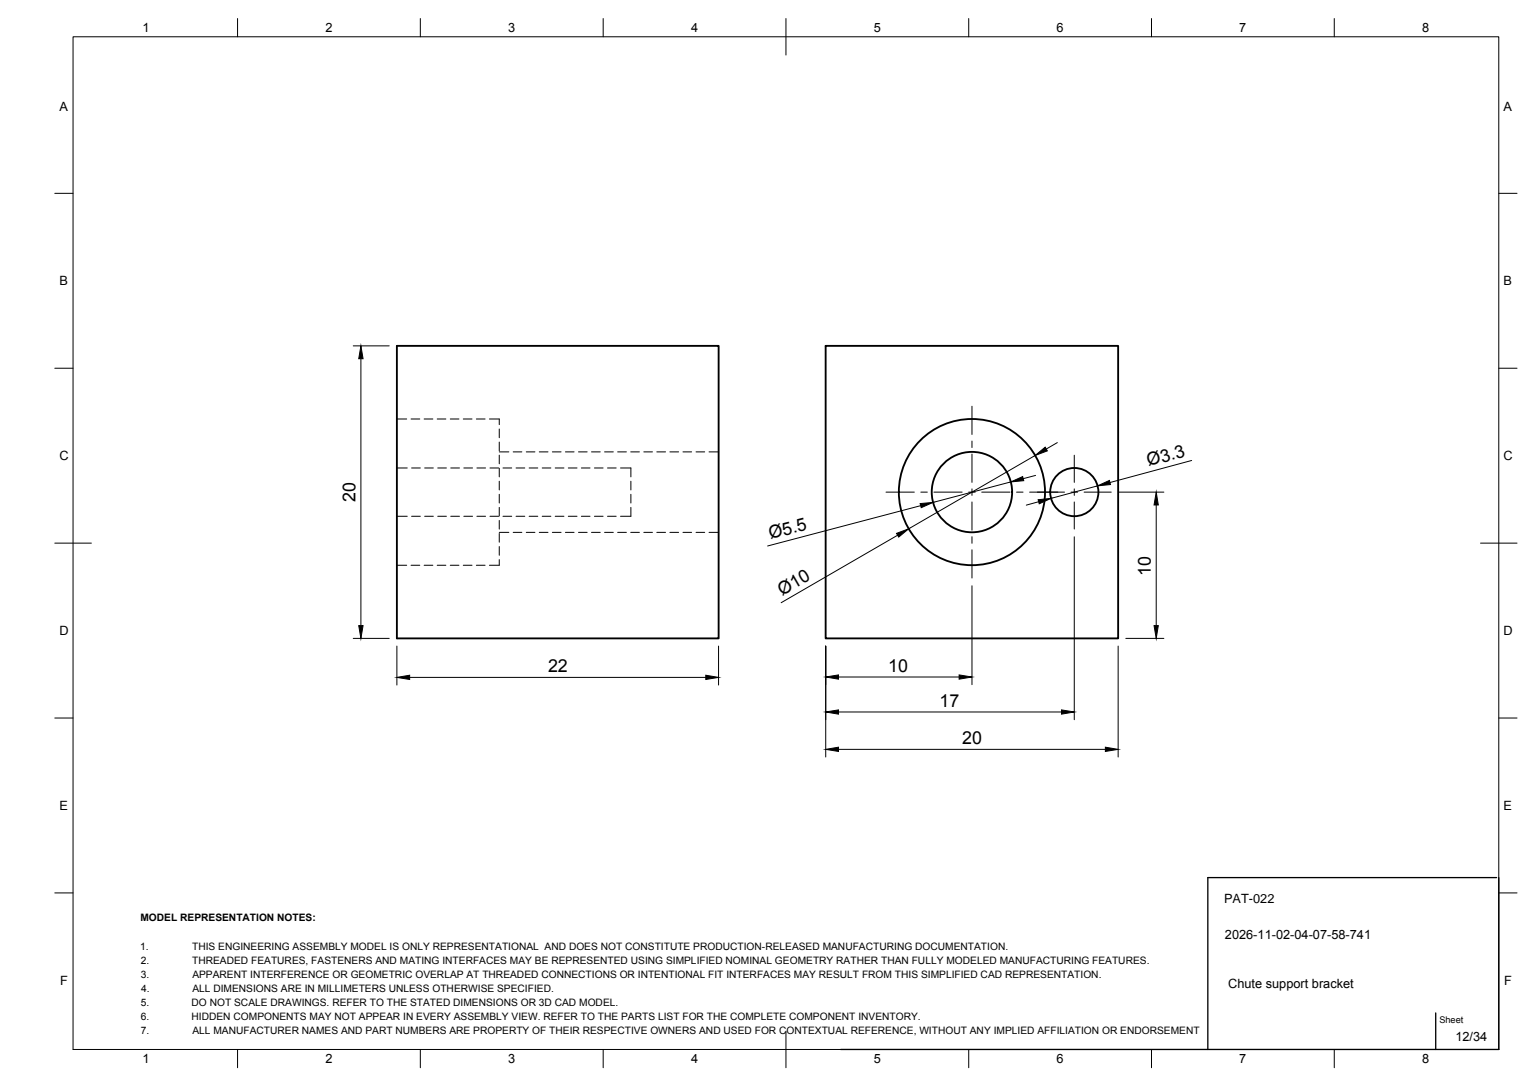
ISO-10303-21;
HEADER;
/* Generated by software containing ST-Developer
 * from STEP Tools, Inc. (www.steptools.com) 
 */

FILE_DESCRIPTION(
/* description */ ('Chute with adjustable gate'),
/* implementation_level */ '2;1');

FILE_NAME(
/* name */ 'Chute support bracket.step',
/* time_stamp */ '2026-10-27T10:52:28-07:00',
/* author */ (''),
/* organization */ (''),
/* preprocessor_version */ 'ST-DEVELOPER v20.2',
/* originating_system */ 'Autodesk Translation Framework v15.17.0.0',
/* authorisation */ '');

FILE_SCHEMA (('AUTOMOTIVE_DESIGN { 1 0 10303 214 3 1 1 }'));
ENDSEC;

DATA;
#10=MECHANICAL_DESIGN_GEOMETRIC_PRESENTATION_REPRESENTATION('',(#421),#13094);
#357=SHAPE_REPRESENTATION_RELATIONSHIP('SRR','None',#13258,#389);
#389=ADVANCED_BREP_SHAPE_REPRESENTATION('',(#453),#13067);
#421=STYLED_ITEM('',(#13474),#453);
#453=MANIFOLD_SOLID_BREP('Body1',#7604);
#500=FACE_BOUND('',#1417,.T.);
#501=FACE_BOUND('',#1420,.T.);
#502=FACE_BOUND('',#1421,.T.);
#503=FACE_BOUND('',#1424,.T.);
#636=PLANE('',#8081);
#637=PLANE('',#8085);
#638=PLANE('',#8089);
#639=PLANE('',#8090);
#640=PLANE('',#8091);
#641=PLANE('',#8092);
#642=PLANE('',#8093);
#643=PLANE('',#8094);
#972=FACE_OUTER_BOUND('',#1413,.T.);
#973=FACE_OUTER_BOUND('',#1414,.T.);
#974=FACE_OUTER_BOUND('',#1415,.T.);
#975=FACE_OUTER_BOUND('',#1416,.T.);
#976=FACE_OUTER_BOUND('',#1418,.T.);
#977=FACE_OUTER_BOUND('',#1419,.T.);
#978=FACE_OUTER_BOUND('',#1422,.T.);
#979=FACE_OUTER_BOUND('',#1423,.T.);
#980=FACE_OUTER_BOUND('',#1425,.T.);
#981=FACE_OUTER_BOUND('',#1426,.T.);
#982=FACE_OUTER_BOUND('',#1427,.T.);
#1413=EDGE_LOOP('',(#5450,#5451,#5452,#5453));
#1414=EDGE_LOOP('',(#5454));
#1415=EDGE_LOOP('',(#5455,#5456,#5457,#5458));
#1416=EDGE_LOOP('',(#5459));
#1417=EDGE_LOOP('',(#5460));
#1418=EDGE_LOOP('',(#5461,#5462,#5463,#5464));
#1419=EDGE_LOOP('',(#5465,#5466,#5467,#5468));
#1420=EDGE_LOOP('',(#5469));
#1421=EDGE_LOOP('',(#5470));
#1422=EDGE_LOOP('',(#5471,#5472,#5473,#5474));
#1423=EDGE_LOOP('',(#5475,#5476,#5477,#5478));
#1424=EDGE_LOOP('',(#5479));
#1425=EDGE_LOOP('',(#5480,#5481,#5482,#5483));
#1426=EDGE_LOOP('',(#5484,#5485,#5486,#5487));
#1427=EDGE_LOOP('',(#5488,#5489,#5490,#5491));
#1968=LINE('',#11191,#2745);
#1969=LINE('',#11198,#2746);
#1970=LINE('',#11206,#2747);
#1971=LINE('',#11210,#2748);
#1972=LINE('',#11212,#2749);
#1973=LINE('',#11214,#2750);
#1974=LINE('',#11215,#2751);
#1975=LINE('',#11218,#2752);
#1976=LINE('',#11220,#2753);
#1977=LINE('',#11221,#2754);
#1978=LINE('',#11224,#2755);
#1979=LINE('',#11226,#2756);
#1980=LINE('',#11227,#2757);
#1981=LINE('',#11229,#2758);
#1982=LINE('',#11230,#2759);
#2745=VECTOR('',#8994,0.165);
#2746=VECTOR('',#9003,0.5);
#2747=VECTOR('',#9014,0.275);
#2748=VECTOR('',#9017,1.);
#2749=VECTOR('',#9018,1.);
#2750=VECTOR('',#9019,1.);
#2751=VECTOR('',#9020,1.);
#2752=VECTOR('',#9023,1.);
#2753=VECTOR('',#9024,1.);
#2754=VECTOR('',#9025,1.);
#2755=VECTOR('',#9028,1.);
#2756=VECTOR('',#9029,1.);
#2757=VECTOR('',#9030,1.);
#2758=VECTOR('',#9033,1.);
#2759=VECTOR('',#9034,1.);
#3438=CIRCLE('',#8079,0.165);
#3439=CIRCLE('',#8080,0.165);
#3440=CIRCLE('',#8083,0.5);
#3441=CIRCLE('',#8084,0.5);
#3442=CIRCLE('',#8086,0.275);
#3443=CIRCLE('',#8088,0.275);
#3681=VERTEX_POINT('',#11188);
#3682=VERTEX_POINT('',#11190);
#3683=VERTEX_POINT('',#11195);
#3684=VERTEX_POINT('',#11197);
#3685=VERTEX_POINT('',#11201);
#3686=VERTEX_POINT('',#11204);
#3687=VERTEX_POINT('',#11208);
#3688=VERTEX_POINT('',#11209);
#3689=VERTEX_POINT('',#11211);
#3690=VERTEX_POINT('',#11213);
#3691=VERTEX_POINT('',#11217);
#3692=VERTEX_POINT('',#11219);
#3693=VERTEX_POINT('',#11223);
#3694=VERTEX_POINT('',#11225);
#4358=EDGE_CURVE('',#3681,#3681,#3438,.T.);
#4359=EDGE_CURVE('',#3681,#3682,#1968,.T.);
#4360=EDGE_CURVE('',#3682,#3682,#3439,.T.);
#4361=EDGE_CURVE('',#3683,#3683,#3440,.T.);
#4362=EDGE_CURVE('',#3683,#3684,#1969,.T.);
#4363=EDGE_CURVE('',#3684,#3684,#3441,.T.);
#4364=EDGE_CURVE('',#3685,#3685,#3442,.T.);
#4365=EDGE_CURVE('',#3686,#3686,#3443,.T.);
#4366=EDGE_CURVE('',#3686,#3685,#1970,.T.);
#4367=EDGE_CURVE('',#3687,#3688,#1971,.T.);
#4368=EDGE_CURVE('',#3688,#3689,#1972,.T.);
#4369=EDGE_CURVE('',#3690,#3689,#1973,.T.);
#4370=EDGE_CURVE('',#3687,#3690,#1974,.T.);
#4371=EDGE_CURVE('',#3691,#3687,#1975,.T.);
#4372=EDGE_CURVE('',#3692,#3690,#1976,.T.);
#4373=EDGE_CURVE('',#3691,#3692,#1977,.T.);
#4374=EDGE_CURVE('',#3693,#3691,#1978,.T.);
#4375=EDGE_CURVE('',#3694,#3692,#1979,.T.);
#4376=EDGE_CURVE('',#3693,#3694,#1980,.T.);
#4377=EDGE_CURVE('',#3688,#3693,#1981,.T.);
#4378=EDGE_CURVE('',#3689,#3694,#1982,.T.);
#5450=ORIENTED_EDGE('',*,*,#4358,.F.);
#5451=ORIENTED_EDGE('',*,*,#4359,.T.);
#5452=ORIENTED_EDGE('',*,*,#4360,.F.);
#5453=ORIENTED_EDGE('',*,*,#4359,.F.);
#5454=ORIENTED_EDGE('',*,*,#4358,.T.);
#5455=ORIENTED_EDGE('',*,*,#4361,.F.);
#5456=ORIENTED_EDGE('',*,*,#4362,.T.);
#5457=ORIENTED_EDGE('',*,*,#4363,.F.);
#5458=ORIENTED_EDGE('',*,*,#4362,.F.);
#5459=ORIENTED_EDGE('',*,*,#4361,.T.);
#5460=ORIENTED_EDGE('',*,*,#4364,.F.);
#5461=ORIENTED_EDGE('',*,*,#4365,.F.);
#5462=ORIENTED_EDGE('',*,*,#4366,.T.);
#5463=ORIENTED_EDGE('',*,*,#4364,.T.);
#5464=ORIENTED_EDGE('',*,*,#4366,.F.);
#5465=ORIENTED_EDGE('',*,*,#4367,.T.);
#5466=ORIENTED_EDGE('',*,*,#4368,.T.);
#5467=ORIENTED_EDGE('',*,*,#4369,.F.);
#5468=ORIENTED_EDGE('',*,*,#4370,.F.);
#5469=ORIENTED_EDGE('',*,*,#4360,.T.);
#5470=ORIENTED_EDGE('',*,*,#4363,.T.);
#5471=ORIENTED_EDGE('',*,*,#4371,.T.);
#5472=ORIENTED_EDGE('',*,*,#4370,.T.);
#5473=ORIENTED_EDGE('',*,*,#4372,.F.);
#5474=ORIENTED_EDGE('',*,*,#4373,.F.);
#5475=ORIENTED_EDGE('',*,*,#4374,.T.);
#5476=ORIENTED_EDGE('',*,*,#4373,.T.);
#5477=ORIENTED_EDGE('',*,*,#4375,.F.);
#5478=ORIENTED_EDGE('',*,*,#4376,.F.);
#5479=ORIENTED_EDGE('',*,*,#4365,.T.);
#5480=ORIENTED_EDGE('',*,*,#4377,.T.);
#5481=ORIENTED_EDGE('',*,*,#4376,.T.);
#5482=ORIENTED_EDGE('',*,*,#4378,.F.);
#5483=ORIENTED_EDGE('',*,*,#4368,.F.);
#5484=ORIENTED_EDGE('',*,*,#4378,.T.);
#5485=ORIENTED_EDGE('',*,*,#4375,.T.);
#5486=ORIENTED_EDGE('',*,*,#4372,.T.);
#5487=ORIENTED_EDGE('',*,*,#4369,.T.);
#5488=ORIENTED_EDGE('',*,*,#4377,.F.);
#5489=ORIENTED_EDGE('',*,*,#4367,.F.);
#5490=ORIENTED_EDGE('',*,*,#4371,.F.);
#5491=ORIENTED_EDGE('',*,*,#4374,.F.);
#7118=CYLINDRICAL_SURFACE('',#8078,0.165);
#7119=CYLINDRICAL_SURFACE('',#8082,0.5);
#7120=CYLINDRICAL_SURFACE('',#8087,0.275);
#7240=ADVANCED_FACE('',(#972),#7118,.F.);
#7241=ADVANCED_FACE('',(#973),#636,.T.);
#7242=ADVANCED_FACE('',(#974),#7119,.F.);
#7243=ADVANCED_FACE('',(#975,#500),#637,.T.);
#7244=ADVANCED_FACE('',(#976),#7120,.F.);
#7245=ADVANCED_FACE('',(#977,#501,#502),#638,.T.);
#7246=ADVANCED_FACE('',(#978),#639,.T.);
#7247=ADVANCED_FACE('',(#979,#503),#640,.T.);
#7248=ADVANCED_FACE('',(#980),#641,.T.);
#7249=ADVANCED_FACE('',(#981),#642,.T.);
#7250=ADVANCED_FACE('',(#982),#643,.F.);
#7604=CLOSED_SHELL('',(#7240,#7241,#7242,#7243,#7244,#7245,#7246,#7247,
#7248,#7249,#7250));
#8077=AXIS2_PLACEMENT_3D('',#11186,#8988,#8989);
#8078=AXIS2_PLACEMENT_3D('',#11187,#8990,#8991);
#8079=AXIS2_PLACEMENT_3D('',#11189,#8992,#8993);
#8080=AXIS2_PLACEMENT_3D('',#11192,#8995,#8996);
#8081=AXIS2_PLACEMENT_3D('',#11193,#8997,#8998);
#8082=AXIS2_PLACEMENT_3D('',#11194,#8999,#9000);
#8083=AXIS2_PLACEMENT_3D('',#11196,#9001,#9002);
#8084=AXIS2_PLACEMENT_3D('',#11199,#9004,#9005);
#8085=AXIS2_PLACEMENT_3D('',#11200,#9006,#9007);
#8086=AXIS2_PLACEMENT_3D('',#11202,#9008,#9009);
#8087=AXIS2_PLACEMENT_3D('',#11203,#9010,#9011);
#8088=AXIS2_PLACEMENT_3D('',#11205,#9012,#9013);
#8089=AXIS2_PLACEMENT_3D('',#11207,#9015,#9016);
#8090=AXIS2_PLACEMENT_3D('',#11216,#9021,#9022);
#8091=AXIS2_PLACEMENT_3D('',#11222,#9026,#9027);
#8092=AXIS2_PLACEMENT_3D('',#11228,#9031,#9032);
#8093=AXIS2_PLACEMENT_3D('',#11231,#9035,#9036);
#8094=AXIS2_PLACEMENT_3D('',#11232,#9037,#9038);
#8988=DIRECTION('axis',(0.,0.,1.));
#8989=DIRECTION('refdir',(1.,0.,0.));
#8990=DIRECTION('center_axis',(0.,1.,0.));
#8991=DIRECTION('ref_axis',(1.,0.,0.));
#8992=DIRECTION('center_axis',(0.,1.,0.));
#8993=DIRECTION('ref_axis',(1.,0.,0.));
#8994=DIRECTION('',(0.,1.,0.));
#8995=DIRECTION('center_axis',(0.,-1.,0.));
#8996=DIRECTION('ref_axis',(1.,0.,0.));
#8997=DIRECTION('center_axis',(0.,1.,0.));
#8998=DIRECTION('ref_axis',(1.,0.,0.));
#8999=DIRECTION('center_axis',(0.,1.,0.));
#9000=DIRECTION('ref_axis',(1.,0.,0.));
#9001=DIRECTION('center_axis',(0.,1.,0.));
#9002=DIRECTION('ref_axis',(1.,0.,0.));
#9003=DIRECTION('',(0.,1.,0.));
#9004=DIRECTION('center_axis',(0.,-1.,0.));
#9005=DIRECTION('ref_axis',(1.,0.,0.));
#9006=DIRECTION('center_axis',(0.,1.,0.));
#9007=DIRECTION('ref_axis',(1.,0.,0.));
#9008=DIRECTION('center_axis',(0.,1.,0.));
#9009=DIRECTION('ref_axis',(1.,0.,0.));
#9010=DIRECTION('center_axis',(0.,1.,0.));
#9011=DIRECTION('ref_axis',(1.,0.,0.));
#9012=DIRECTION('center_axis',(0.,1.,0.));
#9013=DIRECTION('ref_axis',(1.,0.,0.));
#9014=DIRECTION('',(0.,1.,0.));
#9015=DIRECTION('center_axis',(0.,1.,0.));
#9016=DIRECTION('ref_axis',(-1.,0.,0.));
#9017=DIRECTION('',(-1.,0.,0.));
#9018=DIRECTION('',(0.,0.,1.));
#9019=DIRECTION('',(-1.,0.,0.));
#9020=DIRECTION('',(0.,0.,1.));
#9021=DIRECTION('center_axis',(1.,0.,0.));
#9022=DIRECTION('ref_axis',(0.,1.,0.));
#9023=DIRECTION('',(0.,1.,0.));
#9024=DIRECTION('',(0.,1.,0.));
#9025=DIRECTION('',(0.,0.,1.));
#9026=DIRECTION('center_axis',(0.,-1.,0.));
#9027=DIRECTION('ref_axis',(1.,0.,0.));
#9028=DIRECTION('',(1.,0.,0.));
#9029=DIRECTION('',(1.,0.,0.));
#9030=DIRECTION('',(0.,0.,1.));
#9031=DIRECTION('center_axis',(-1.,0.,0.));
#9032=DIRECTION('ref_axis',(0.,-1.,0.));
#9033=DIRECTION('',(0.,-1.,0.));
#9034=DIRECTION('',(0.,-1.,0.));
#9035=DIRECTION('center_axis',(0.,0.,1.));
#9036=DIRECTION('ref_axis',(1.,0.,0.));
#9037=DIRECTION('center_axis',(0.,0.,1.));
#9038=DIRECTION('ref_axis',(1.,0.,0.));
#11186=CARTESIAN_POINT('',(0.,0.,0.));
#11187=CARTESIAN_POINT('Origin',(2.3,-9.4,7.));
#11188=CARTESIAN_POINT('',(2.135,-9.4,7.));
#11189=CARTESIAN_POINT('Origin',(2.3,-9.4,7.));
#11190=CARTESIAN_POINT('',(2.135,-7.8,7.));
#11191=CARTESIAN_POINT('',(2.135,-9.4,7.));
#11192=CARTESIAN_POINT('Origin',(2.3,-7.8,7.));
#11193=CARTESIAN_POINT('Origin',(2.3,-9.4,7.));
#11194=CARTESIAN_POINT('Origin',(3.,-8.5,7.));
#11195=CARTESIAN_POINT('',(2.5,-8.5,7.));
#11196=CARTESIAN_POINT('Origin',(3.,-8.5,7.));
#11197=CARTESIAN_POINT('',(2.5,-7.8,7.));
#11198=CARTESIAN_POINT('',(2.5,-8.5,7.));
#11199=CARTESIAN_POINT('Origin',(3.,-7.8,7.));
#11200=CARTESIAN_POINT('Origin',(3.,-8.5,7.));
#11201=CARTESIAN_POINT('',(2.725,-8.5,7.));
#11202=CARTESIAN_POINT('Origin',(3.,-8.5,7.));
#11203=CARTESIAN_POINT('Origin',(3.,-10.1,7.));
#11204=CARTESIAN_POINT('',(2.725,-10.,7.));
#11205=CARTESIAN_POINT('Origin',(3.,-10.,7.));
#11206=CARTESIAN_POINT('',(2.725,-10.1,7.));
#11207=CARTESIAN_POINT('Origin',(4.,-7.8,6.));
#11208=CARTESIAN_POINT('',(4.,-7.8,6.));
#11209=CARTESIAN_POINT('',(2.,-7.8,6.));
#11210=CARTESIAN_POINT('',(4.,-7.8,6.));
#11211=CARTESIAN_POINT('',(2.,-7.8,8.));
#11212=CARTESIAN_POINT('',(2.,-7.8,6.));
#11213=CARTESIAN_POINT('',(4.,-7.8,8.));
#11214=CARTESIAN_POINT('',(4.,-7.8,8.));
#11215=CARTESIAN_POINT('',(4.,-7.8,6.));
#11216=CARTESIAN_POINT('Origin',(4.,-10.,6.));
#11217=CARTESIAN_POINT('',(4.,-10.,6.));
#11218=CARTESIAN_POINT('',(4.,-10.,6.));
#11219=CARTESIAN_POINT('',(4.,-10.,8.));
#11220=CARTESIAN_POINT('',(4.,-10.,8.));
#11221=CARTESIAN_POINT('',(4.,-10.,6.));
#11222=CARTESIAN_POINT('Origin',(2.,-10.,6.));
#11223=CARTESIAN_POINT('',(2.,-10.,6.));
#11224=CARTESIAN_POINT('',(2.,-10.,6.));
#11225=CARTESIAN_POINT('',(2.,-10.,8.));
#11226=CARTESIAN_POINT('',(2.,-10.,8.));
#11227=CARTESIAN_POINT('',(2.,-10.,6.));
#11228=CARTESIAN_POINT('Origin',(2.,-7.8,6.));
#11229=CARTESIAN_POINT('',(2.,-7.8,6.));
#11230=CARTESIAN_POINT('',(2.,-7.8,8.));
#11231=CARTESIAN_POINT('Origin',(3.,-8.9,8.));
#11232=CARTESIAN_POINT('Origin',(3.,-8.9,6.));
#13030=UNCERTAINTY_MEASURE_WITH_UNIT(LENGTH_MEASURE(0.001),#13095,
'DISTANCE_ACCURACY_VALUE',
'Maximum model space distance between geometric entities at asserted c
onnectivities');
#13057=UNCERTAINTY_MEASURE_WITH_UNIT(LENGTH_MEASURE(0.001),#13095,
'DISTANCE_ACCURACY_VALUE',
'Maximum model space distance between geometric entities at asserted c
onnectivities');
#13067=(
GEOMETRIC_REPRESENTATION_CONTEXT(3)
GLOBAL_UNCERTAINTY_ASSIGNED_CONTEXT((#13030))
GLOBAL_UNIT_ASSIGNED_CONTEXT((#13095,#13097,#13098))
REPRESENTATION_CONTEXT('','3D')
);
#13094=(
GEOMETRIC_REPRESENTATION_CONTEXT(3)
GLOBAL_UNCERTAINTY_ASSIGNED_CONTEXT((#13057))
GLOBAL_UNIT_ASSIGNED_CONTEXT((#13095,#13097,#13098))
REPRESENTATION_CONTEXT('','3D')
);
#13095=(
LENGTH_UNIT()
NAMED_UNIT(*)
SI_UNIT(.CENTI.,.METRE.)
);
#13097=(
NAMED_UNIT(*)
PLANE_ANGLE_UNIT()
SI_UNIT($,.RADIAN.)
);
#13098=(
NAMED_UNIT(*)
SI_UNIT($,.STERADIAN.)
SOLID_ANGLE_UNIT()
);
#13108=SHAPE_DEFINITION_REPRESENTATION(#13144,#13258);
#13144=PRODUCT_DEFINITION_SHAPE('',$,#13295);
#13258=SHAPE_REPRESENTATION('',(#8077),#13067);
#13285=PRODUCT_DEFINITION_CONTEXT('part definition',#13395,'design');
#13295=PRODUCT_DEFINITION('Chute support bracket',
'Chute support bracket',#13331,#13285);
#13331=PRODUCT_DEFINITION_FORMATION('',$,#13406);
#13395=APPLICATION_CONTEXT(
'Core Data for Automotive Mechanical Design Process');
#13396=PRODUCT_CONTEXT('part definition',#13395,'mechanical');
#13406=PRODUCT('Chute support bracket','Chute support bracket',
'Chute support bracket',(#13396));
#13468=COLOUR_RGB('Dark Blue',0.08,0.2,0.34);
#13469=FILL_AREA_STYLE_COLOUR('',#13468);
#13470=FILL_AREA_STYLE('',(#13469));
#13471=SURFACE_STYLE_FILL_AREA(#13470);
#13472=SURFACE_SIDE_STYLE('',(#13471));
#13473=SURFACE_STYLE_USAGE(.BOTH.,#13472);
#13474=PRESENTATION_STYLE_ASSIGNMENT((#13473));
ENDSEC;
END-ISO-10303-21;
